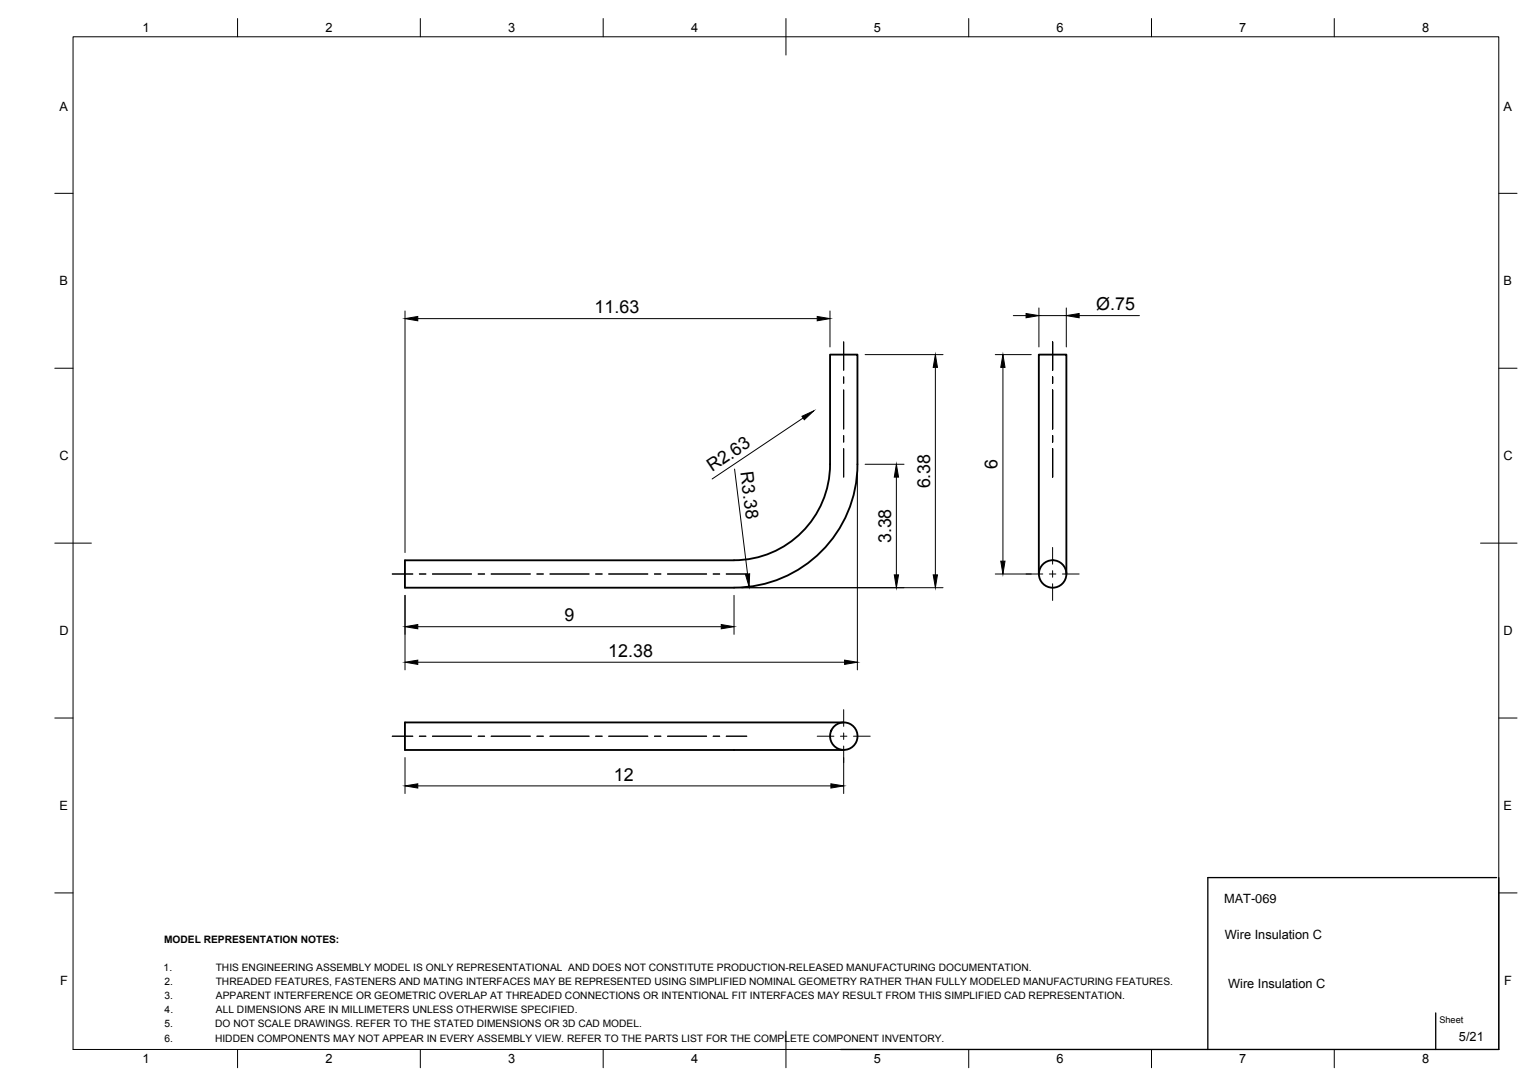
ISO-10303-21;
HEADER;
/* Generated by software containing ST-Developer
 * from STEP Tools, Inc. (www.steptools.com) 
 */

FILE_DESCRIPTION(
/* description */ ('CAx-IF Rec.Pracs.---Representation and Presentation of Product Manufa
cturing Information (PMI)---4.0---2014-10-13'),
/* implementation_level */ '2;1');

FILE_NAME(
/* name */ 'Wire Insulation C.step',
/* time_stamp */ '2026-10-24T15:08:39-07:00',
/* author */ (''),
/* organization */ (''),
/* preprocessor_version */ 'ST-DEVELOPER v20.2',
/* originating_system */ 'Autodesk Translation Framework v15.17.0.0',
/* authorisation */ '');

FILE_SCHEMA (('AP242_MANAGED_MODEL_BASED_3D_ENGINEERING_MIM_LF { 1 0 10303 442 2 1 4 }'));
ENDSEC;

DATA;
#10=MECHANICAL_DESIGN_GEOMETRIC_PRESENTATION_REPRESENTATION('',(#822),#50081);
#770=TOROIDAL_SURFACE('',#10133,0.003,0.000375);
#782=SHAPE_REPRESENTATION_RELATIONSHIP('SRR','None',#50150,#802);
#802=ADVANCED_BREP_SHAPE_REPRESENTATION('',(#842),#50063);
#822=STYLED_ITEM('',(#50259),#842);
#842=MANIFOLD_SOLID_BREP('Body1',#9867);
#864=PLANE('',#10127);
#865=PLANE('',#10138);
#1110=FACE_OUTER_BOUND('',#1651,.T.);
#1111=FACE_OUTER_BOUND('',#1652,.T.);
#1112=FACE_OUTER_BOUND('',#1653,.T.);
#1113=FACE_OUTER_BOUND('',#1654,.T.);
#1114=FACE_OUTER_BOUND('',#1655,.T.);
#1651=EDGE_LOOP('',(#6250));
#1652=EDGE_LOOP('',(#6251,#6252,#6253,#6254,#6255));
#1653=EDGE_LOOP('',(#6256,#6257,#6258,#6259,#6260,#6261));
#1654=EDGE_LOOP('',(#6262,#6263,#6264,#6265,#6266));
#1655=EDGE_LOOP('',(#6267));
#2246=LINE('',#13510,#2824);
#2247=LINE('',#13521,#2825);
#2824=VECTOR('',#11088,0.000375);
#2825=VECTOR('',#11103,0.000375);
#3408=CIRCLE('',#10128,0.00037500000001);
#3409=CIRCLE('',#10130,0.00037500000001);
#3410=CIRCLE('',#10131,0.00037500000001);
#3411=CIRCLE('',#10132,0.00037500000001);
#3412=CIRCLE('',#10134,0.002625);
#3413=CIRCLE('',#10135,0.00037500000001);
#3414=CIRCLE('',#10136,0.00037500000001);
#3780=VERTEX_POINT('',#13504);
#3781=VERTEX_POINT('',#13507);
#3782=VERTEX_POINT('',#13509);
#3783=VERTEX_POINT('',#13511);
#3784=VERTEX_POINT('',#13515);
#3785=VERTEX_POINT('',#13517);
#4778=EDGE_CURVE('',#3780,#3780,#3408,.T.);
#4779=EDGE_CURVE('',#3781,#3781,#3409,.T.);
#4780=EDGE_CURVE('',#3781,#3782,#2246,.T.);
#4781=EDGE_CURVE('',#3782,#3783,#3410,.T.);
#4782=EDGE_CURVE('',#3783,#3782,#3411,.T.);
#4783=EDGE_CURVE('',#3783,#3784,#3412,.T.);
#4784=EDGE_CURVE('',#3784,#3785,#3413,.T.);
#4785=EDGE_CURVE('',#3785,#3784,#3414,.T.);
#4786=EDGE_CURVE('',#3785,#3780,#2247,.T.);
#6250=ORIENTED_EDGE('',*,*,#4778,.F.);
#6251=ORIENTED_EDGE('',*,*,#4779,.F.);
#6252=ORIENTED_EDGE('',*,*,#4780,.T.);
#6253=ORIENTED_EDGE('',*,*,#4781,.T.);
#6254=ORIENTED_EDGE('',*,*,#4782,.T.);
#6255=ORIENTED_EDGE('',*,*,#4780,.F.);
#6256=ORIENTED_EDGE('',*,*,#4782,.F.);
#6257=ORIENTED_EDGE('',*,*,#4783,.T.);
#6258=ORIENTED_EDGE('',*,*,#4784,.T.);
#6259=ORIENTED_EDGE('',*,*,#4785,.T.);
#6260=ORIENTED_EDGE('',*,*,#4783,.F.);
#6261=ORIENTED_EDGE('',*,*,#4781,.F.);
#6262=ORIENTED_EDGE('',*,*,#4785,.F.);
#6263=ORIENTED_EDGE('',*,*,#4786,.T.);
#6264=ORIENTED_EDGE('',*,*,#4778,.T.);
#6265=ORIENTED_EDGE('',*,*,#4786,.F.);
#6266=ORIENTED_EDGE('',*,*,#4784,.F.);
#6267=ORIENTED_EDGE('',*,*,#4779,.T.);
#9149=CYLINDRICAL_SURFACE('',#10129,0.000375);
#9150=CYLINDRICAL_SURFACE('',#10137,0.000375);
#9332=ADVANCED_FACE('',(#1110),#864,.F.);
#9333=ADVANCED_FACE('',(#1111),#9149,.T.);
#9334=ADVANCED_FACE('',(#1112),#770,.T.);
#9335=ADVANCED_FACE('',(#1113),#9150,.T.);
#9336=ADVANCED_FACE('',(#1114),#865,.T.);
#9867=CLOSED_SHELL('',(#9332,#9333,#9334,#9335,#9336));
#10126=AXIS2_PLACEMENT_3D('',#13502,#11078,#11079);
#10127=AXIS2_PLACEMENT_3D('',#13503,#11080,#11081);
#10128=AXIS2_PLACEMENT_3D('',#13505,#11082,#11083);
#10129=AXIS2_PLACEMENT_3D('',#13506,#11084,#11085);
#10130=AXIS2_PLACEMENT_3D('',#13508,#11086,#11087);
#10131=AXIS2_PLACEMENT_3D('',#13512,#11089,#11090);
#10132=AXIS2_PLACEMENT_3D('',#13513,#11091,#11092);
#10133=AXIS2_PLACEMENT_3D('',#13514,#11093,#11094);
#10134=AXIS2_PLACEMENT_3D('',#13516,#11095,#11096);
#10135=AXIS2_PLACEMENT_3D('',#13518,#11097,#11098);
#10136=AXIS2_PLACEMENT_3D('',#13519,#11099,#11100);
#10137=AXIS2_PLACEMENT_3D('',#13520,#11101,#11102);
#10138=AXIS2_PLACEMENT_3D('',#13522,#11104,#11105);
#11078=DIRECTION('axis',(0.,0.,1.));
#11079=DIRECTION('refdir',(1.,0.,0.));
#11080=DIRECTION('center_axis',(0.906307787036647,-0.422618261740706,-8.00429517722823E-16));
#11081=DIRECTION('ref_axis',(2.42833204006769E-16,2.41473507855972E-15,
-1.));
#11082=DIRECTION('center_axis',(0.906307787036647,-0.422618261740706,-8.00429517722823E-16));
#11083=DIRECTION('ref_axis',(0.422618261740706,0.906307787036647,1.97116866169388E-15));
#11084=DIRECTION('center_axis',(2.42833204006769E-16,2.41473507855972E-15,
-1.));
#11085=DIRECTION('ref_axis',(0.422618261740706,0.906307787036647,2.29111895189949E-15));
#11086=DIRECTION('center_axis',(2.41685059822166E-11,-1.12674314556115E-11,
-1.));
#11087=DIRECTION('ref_axis',(0.422618261740706,0.906307787036647,2.29111895186703E-15));
#11088=DIRECTION('',(-2.42833204006769E-16,-2.41473507855972E-15,1.));
#11089=DIRECTION('center_axis',(2.41685059822166E-11,-1.12674314556115E-11,
-1.));
#11090=DIRECTION('ref_axis',(0.422618261740706,0.906307787036647,2.29111895186703E-15));
#11091=DIRECTION('center_axis',(2.41685059822166E-11,-1.12674314556115E-11,
-1.));
#11092=DIRECTION('ref_axis',(0.422618261740706,0.906307787036647,2.29111895186703E-15));
#11093=DIRECTION('center_axis',(0.422618261740706,0.906307787036647,1.97116866169388E-15));
#11094=DIRECTION('ref_axis',(1.28498035257541E-16,2.05596856412066E-15,
-1.));
#11095=DIRECTION('center_axis',(-0.422618261740706,-0.906307787036647,-1.97116866169388E-15));
#11096=DIRECTION('ref_axis',(3.58767987664542E-16,2.00764771571504E-15,
-1.));
#11097=DIRECTION('center_axis',(0.906307787036647,-0.422618261740706,-8.00429517722823E-16));
#11098=DIRECTION('ref_axis',(0.422618261740706,0.906307787036647,1.97116866169388E-15));
#11099=DIRECTION('center_axis',(0.906307787036647,-0.422618261740706,-8.00429517722823E-16));
#11100=DIRECTION('ref_axis',(0.422618261740706,0.906307787036647,1.97116866169388E-15));
#11101=DIRECTION('center_axis',(0.906307787036647,-0.422618261740706,-8.00429517722823E-16));
#11102=DIRECTION('ref_axis',(0.422618261740706,0.906307787036647,1.97116866169388E-15));
#11103=DIRECTION('',(-0.906307787036647,0.422618261740706,8.00429517722823E-16));
#11104=DIRECTION('center_axis',(2.98328550528607E-16,2.38885717348462E-15,
-1.));
#11105=DIRECTION('ref_axis',(0.906307787036647,-0.422618261740706,-7.39197177765454E-16));
#13502=CARTESIAN_POINT('',(0.,0.,0.));
#13503=CARTESIAN_POINT('Origin',(-0.00466438431356942,-0.0300042013554656,
0.00162414671344191));
#13504=CARTESIAN_POINT('',(-0.00482286616173126,-0.0303440667756001,0.0016241467134419));
#13505=CARTESIAN_POINT('Origin',(-0.00466438431357425,-0.0300042013554523,
0.00162414671345191));
#13506=CARTESIAN_POINT('Origin',(0.00621130913087035,-0.035075620496354,
-0.0013758532865581));
#13507=CARTESIAN_POINT('',(0.00605282728271759,-0.0354154859164927,-0.0043758532865581));
#13508=CARTESIAN_POINT('Origin',(0.00621130913087458,-0.035075620496345,
-0.0043758532865481));
#13509=CARTESIAN_POINT('',(0.00605282728271759,-0.0354154859164927,-0.0013758532865381));
#13510=CARTESIAN_POINT('',(0.00605282728271759,-0.0354154859164927,-0.0013758532865581));
#13511=CARTESIAN_POINT('',(0.00587144371072257,-0.034917138648197,-0.0013758532865581));
#13512=CARTESIAN_POINT('Origin',(0.00621130913087458,-0.035075620496345,
-0.0013758532865481));
#13513=CARTESIAN_POINT('Origin',(0.00621130913087458,-0.035075620496345,
-0.0013758532865481));
#13514=CARTESIAN_POINT('Origin',(0.00349238576976041,-0.0338077657111319,
-0.0013758532865581));
#13515=CARTESIAN_POINT('',(0.00349238576975134,-0.0338077657111277,0.0012491467134419));
#13516=CARTESIAN_POINT('Origin',(0.00349238576976041,-0.0338077657111319,
-0.0013758532865581));
#13517=CARTESIAN_POINT('',(0.00333390392159855,-0.0341476311312665,0.0016241467134419));
#13518=CARTESIAN_POINT('Origin',(0.00349238576975557,-0.0338077657111186,
0.0016241467134519));
#13519=CARTESIAN_POINT('Origin',(0.00349238576975557,-0.0338077657111186,
0.0016241467134519));
#13520=CARTESIAN_POINT('Origin',(-0.0101022310357893,-0.0274684917850214,
0.00162414671344191));
#13521=CARTESIAN_POINT('',(-0.0102607128839421,-0.0278083572051601,0.00162414671344191));
#13522=CARTESIAN_POINT('Origin',(0.00621130913087035,-0.035075620496354,
-0.0043758532865581));
#50041=UNCERTAINTY_MEASURE_WITH_UNIT(LENGTH_MEASURE(1.E-5),#50082,
'DISTANCE_ACCURACY_VALUE',
'Maximum model space distance between geometric entities at asserted c
onnectivities');
#50059=UNCERTAINTY_MEASURE_WITH_UNIT(LENGTH_MEASURE(1.E-5),#50082,
'DISTANCE_ACCURACY_VALUE',
'Maximum model space distance between geometric entities at asserted c
onnectivities');
#50063=(
GEOMETRIC_REPRESENTATION_CONTEXT(3)
GLOBAL_UNCERTAINTY_ASSIGNED_CONTEXT((#50041))
GLOBAL_UNIT_ASSIGNED_CONTEXT((#50082,#50083,#50084))
REPRESENTATION_CONTEXT('','3D')
);
#50081=(
GEOMETRIC_REPRESENTATION_CONTEXT(3)
GLOBAL_UNCERTAINTY_ASSIGNED_CONTEXT((#50059))
GLOBAL_UNIT_ASSIGNED_CONTEXT((#50082,#50083,#50084))
REPRESENTATION_CONTEXT('','3D')
);
#50082=(
LENGTH_UNIT()
NAMED_UNIT(*)
SI_UNIT($,.METRE.)
);
#50083=(
NAMED_UNIT(*)
PLANE_ANGLE_UNIT()
SI_UNIT($,.RADIAN.)
);
#50084=(
NAMED_UNIT(*)
SI_UNIT($,.STERADIAN.)
SOLID_ANGLE_UNIT()
);
#50088=SHAPE_DEFINITION_REPRESENTATION(#50109,#50150);
#50109=PRODUCT_DEFINITION_SHAPE('',$,#50172);
#50150=SHAPE_REPRESENTATION('',(#10126),#50063);
#50168=PRODUCT_DEFINITION_CONTEXT('part definition',#50233,'design');
#50172=PRODUCT_DEFINITION('Wire Insulation C','Wire Insulation C',#50193,
#50168);
#50193=PRODUCT_DEFINITION_FORMATION('',$,#50238);
#50233=APPLICATION_CONTEXT('Managed model based 3d engineering');
#50234=PRODUCT_CONTEXT('part definition',#50233,'mechanical');
#50238=PRODUCT('Wire Insulation C','Wire Insulation C',
'Sensor Cartridge v1',(#50234));
#50259=PRESENTATION_STYLE_ASSIGNMENT((#50266));
#50266=SURFACE_STYLE_USAGE(.BOTH.,#50273);
#50273=SURFACE_SIDE_STYLE('',(#50280));
#50280=SURFACE_STYLE_FILL_AREA(#50287);
#50287=FILL_AREA_STYLE('Opaque(246,246,243)',(#50294));
#50294=FILL_AREA_STYLE_COLOUR('Opaque(246,246,243)',#50301);
#50301=COLOUR_RGB('Opaque(246,246,243)',0.964705882352941,0.964705882352941,
0.952941176470588);
ENDSEC;
END-ISO-10303-21;
